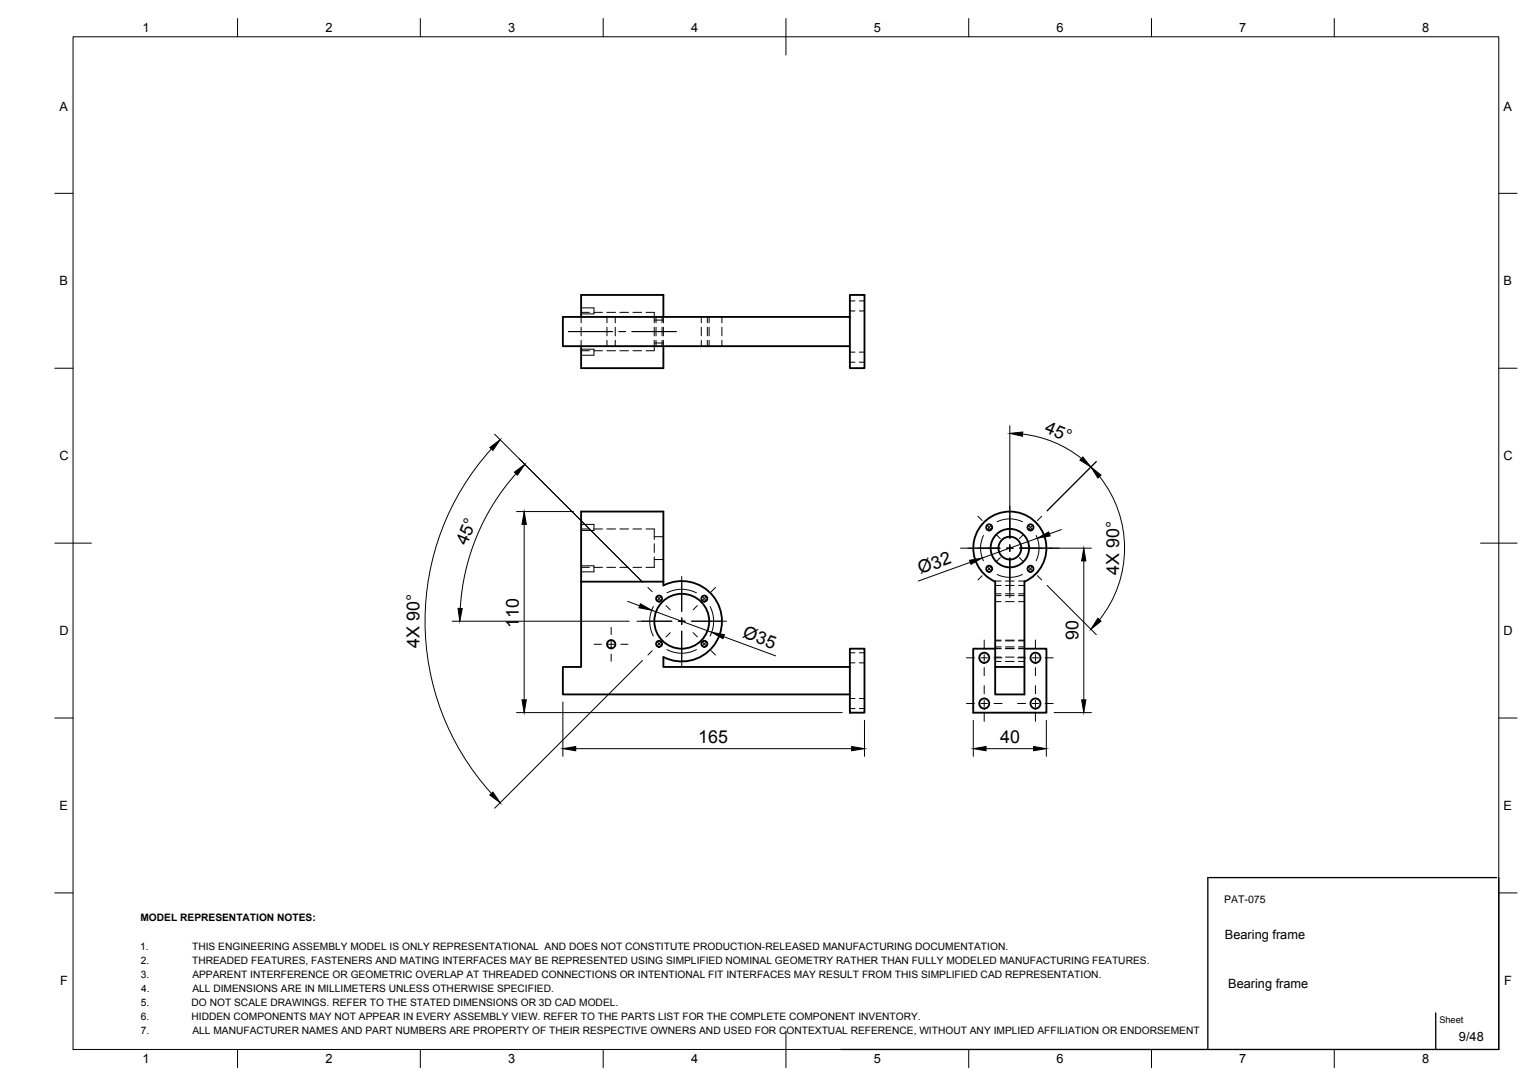
ISO-10303-21;
HEADER;
/* Generated by software containing ST-Developer
 * from STEP Tools, Inc. (www.steptools.com) 
 */

FILE_DESCRIPTION(
/* description */ ('Over-Centre Plunger Toggle Clamp on Slotted Fixture Frame'),
/* implementation_level */ '2;1');

FILE_NAME(
/* name */ 
'Bearing frame.step',
/* time_stamp */ '2026-10-28T03:23:24-07:00',
/* author */ (''),
/* organization */ (''),
/* preprocessor_version */ 'ST-DEVELOPER v20.2',
/* originating_system */ 'Autodesk Translation Framework v15.17.0.0',
/* authorisation */ '');

FILE_SCHEMA (('AUTOMOTIVE_DESIGN { 1 0 10303 214 3 1 1 }'));
ENDSEC;

DATA;
#10=MECHANICAL_DESIGN_GEOMETRIC_PRESENTATION_REPRESENTATION('',(#517),#15212);
#433=SHAPE_REPRESENTATION_RELATIONSHIP('SRR','None',#15407,#475);
#475=ADVANCED_BREP_SHAPE_REPRESENTATION('',(#568),#15169);
#517=STYLED_ITEM('',(#15719),#568);
#568=MANIFOLD_SOLID_BREP('Body1',#8249);
#643=FACE_BOUND('',#1664,.T.);
#644=FACE_BOUND('',#1669,.T.);
#645=FACE_BOUND('',#1670,.T.);
#646=FACE_BOUND('',#1671,.T.);
#647=FACE_BOUND('',#1672,.T.);
#648=FACE_BOUND('',#1673,.T.);
#649=FACE_BOUND('',#1674,.T.);
#650=FACE_BOUND('',#1676,.T.);
#651=FACE_BOUND('',#1677,.T.);
#652=FACE_BOUND('',#1678,.T.);
#653=FACE_BOUND('',#1679,.T.);
#654=FACE_BOUND('',#1680,.T.);
#655=FACE_BOUND('',#1682,.T.);
#656=FACE_BOUND('',#1683,.T.);
#657=FACE_BOUND('',#1684,.T.);
#658=FACE_BOUND('',#1685,.T.);
#659=FACE_BOUND('',#1686,.T.);
#660=FACE_BOUND('',#1694,.T.);
#661=FACE_BOUND('',#1695,.T.);
#662=FACE_BOUND('',#1696,.T.);
#663=FACE_BOUND('',#1697,.T.);
#664=FACE_BOUND('',#1698,.T.);
#665=FACE_BOUND('',#1699,.T.);
#666=FACE_BOUND('',#1702,.T.);
#667=FACE_BOUND('',#1707,.T.);
#668=FACE_BOUND('',#1708,.T.);
#669=FACE_BOUND('',#1709,.T.);
#670=FACE_BOUND('',#1710,.T.);
#807=PLANE('',#8848);
#808=PLANE('',#8852);
#809=PLANE('',#8856);
#810=PLANE('',#8860);
#811=PLANE('',#8888);
#812=PLANE('',#8898);
#813=PLANE('',#8900);
#814=PLANE('',#8901);
#815=PLANE('',#8902);
#816=PLANE('',#8903);
#817=PLANE('',#8904);
#818=PLANE('',#8905);
#819=PLANE('',#8906);
#820=PLANE('',#8909);
#821=PLANE('',#8910);
#822=PLANE('',#8911);
#823=PLANE('',#8912);
#824=PLANE('',#8913);
#825=PLANE('',#8914);
#826=PLANE('',#8915);
#1127=FACE_OUTER_BOUND('',#1645,.T.);
#1128=FACE_OUTER_BOUND('',#1646,.T.);
#1129=FACE_OUTER_BOUND('',#1647,.T.);
#1130=FACE_OUTER_BOUND('',#1648,.T.);
#1131=FACE_OUTER_BOUND('',#1649,.T.);
#1132=FACE_OUTER_BOUND('',#1650,.T.);
#1133=FACE_OUTER_BOUND('',#1651,.T.);
#1134=FACE_OUTER_BOUND('',#1652,.T.);
#1135=FACE_OUTER_BOUND('',#1653,.T.);
#1136=FACE_OUTER_BOUND('',#1654,.T.);
#1137=FACE_OUTER_BOUND('',#1655,.T.);
#1138=FACE_OUTER_BOUND('',#1656,.T.);
#1139=FACE_OUTER_BOUND('',#1657,.T.);
#1140=FACE_OUTER_BOUND('',#1658,.T.);
#1141=FACE_OUTER_BOUND('',#1659,.T.);
#1142=FACE_OUTER_BOUND('',#1660,.T.);
#1143=FACE_OUTER_BOUND('',#1661,.T.);
#1144=FACE_OUTER_BOUND('',#1662,.T.);
#1145=FACE_OUTER_BOUND('',#1663,.T.);
#1146=FACE_OUTER_BOUND('',#1665,.T.);
#1147=FACE_OUTER_BOUND('',#1666,.T.);
#1148=FACE_OUTER_BOUND('',#1667,.T.);
#1149=FACE_OUTER_BOUND('',#1668,.T.);
#1150=FACE_OUTER_BOUND('',#1675,.T.);
#1151=FACE_OUTER_BOUND('',#1681,.T.);
#1152=FACE_OUTER_BOUND('',#1687,.T.);
#1153=FACE_OUTER_BOUND('',#1688,.T.);
#1154=FACE_OUTER_BOUND('',#1689,.T.);
#1155=FACE_OUTER_BOUND('',#1690,.T.);
#1156=FACE_OUTER_BOUND('',#1691,.T.);
#1157=FACE_OUTER_BOUND('',#1692,.T.);
#1158=FACE_OUTER_BOUND('',#1693,.T.);
#1159=FACE_OUTER_BOUND('',#1700,.T.);
#1160=FACE_OUTER_BOUND('',#1701,.T.);
#1161=FACE_OUTER_BOUND('',#1703,.T.);
#1162=FACE_OUTER_BOUND('',#1704,.T.);
#1163=FACE_OUTER_BOUND('',#1705,.T.);
#1164=FACE_OUTER_BOUND('',#1706,.T.);
#1645=EDGE_LOOP('',(#5761,#5762,#5763,#5764));
#1646=EDGE_LOOP('',(#5765,#5766,#5767,#5768));
#1647=EDGE_LOOP('',(#5769));
#1648=EDGE_LOOP('',(#5770,#5771,#5772,#5773));
#1649=EDGE_LOOP('',(#5774));
#1650=EDGE_LOOP('',(#5775,#5776,#5777,#5778));
#1651=EDGE_LOOP('',(#5779));
#1652=EDGE_LOOP('',(#5780,#5781,#5782,#5783));
#1653=EDGE_LOOP('',(#5784));
#1654=EDGE_LOOP('',(#5785,#5786,#5787,#5788));
#1655=EDGE_LOOP('',(#5789,#5790,#5791,#5792));
#1656=EDGE_LOOP('',(#5793,#5794,#5795,#5796));
#1657=EDGE_LOOP('',(#5797,#5798,#5799,#5800));
#1658=EDGE_LOOP('',(#5801,#5802,#5803,#5804));
#1659=EDGE_LOOP('',(#5805,#5806,#5807,#5808));
#1660=EDGE_LOOP('',(#5809,#5810,#5811,#5812));
#1661=EDGE_LOOP('',(#5813,#5814,#5815,#5816));
#1662=EDGE_LOOP('',(#5817,#5818,#5819,#5820));
#1663=EDGE_LOOP('',(#5821));
#1664=EDGE_LOOP('',(#5822));
#1665=EDGE_LOOP('',(#5823,#5824,#5825,#5826));
#1666=EDGE_LOOP('',(#5827,#5828,#5829,#5830));
#1667=EDGE_LOOP('',(#5831,#5832,#5833,#5834));
#1668=EDGE_LOOP('',(#5835,#5836,#5837,#5838,#5839,#5840,#5841,#5842,#5843,
#5844));
#1669=EDGE_LOOP('',(#5845));
#1670=EDGE_LOOP('',(#5846));
#1671=EDGE_LOOP('',(#5847));
#1672=EDGE_LOOP('',(#5848));
#1673=EDGE_LOOP('',(#5849));
#1674=EDGE_LOOP('',(#5850));
#1675=EDGE_LOOP('',(#5851,#5852,#5853,#5854));
#1676=EDGE_LOOP('',(#5855));
#1677=EDGE_LOOP('',(#5856));
#1678=EDGE_LOOP('',(#5857));
#1679=EDGE_LOOP('',(#5858));
#1680=EDGE_LOOP('',(#5859));
#1681=EDGE_LOOP('',(#5860,#5861,#5862,#5863));
#1682=EDGE_LOOP('',(#5864,#5865,#5866,#5867));
#1683=EDGE_LOOP('',(#5868));
#1684=EDGE_LOOP('',(#5869));
#1685=EDGE_LOOP('',(#5870));
#1686=EDGE_LOOP('',(#5871));
#1687=EDGE_LOOP('',(#5872,#5873,#5874,#5875));
#1688=EDGE_LOOP('',(#5876,#5877,#5878,#5879));
#1689=EDGE_LOOP('',(#5880,#5881,#5882,#5883));
#1690=EDGE_LOOP('',(#5884,#5885,#5886,#5887));
#1691=EDGE_LOOP('',(#5888,#5889,#5890,#5891));
#1692=EDGE_LOOP('',(#5892,#5893,#5894,#5895));
#1693=EDGE_LOOP('',(#5896,#5897,#5898,#5899,#5900,#5901,#5902,#5903,#5904,
#5905));
#1694=EDGE_LOOP('',(#5906));
#1695=EDGE_LOOP('',(#5907));
#1696=EDGE_LOOP('',(#5908));
#1697=EDGE_LOOP('',(#5909));
#1698=EDGE_LOOP('',(#5910));
#1699=EDGE_LOOP('',(#5911));
#1700=EDGE_LOOP('',(#5912,#5913,#5914,#5915));
#1701=EDGE_LOOP('',(#5916,#5917,#5918,#5919));
#1702=EDGE_LOOP('',(#5920));
#1703=EDGE_LOOP('',(#5921,#5922,#5923,#5924));
#1704=EDGE_LOOP('',(#5925,#5926,#5927,#5928));
#1705=EDGE_LOOP('',(#5929,#5930,#5931,#5932));
#1706=EDGE_LOOP('',(#5933,#5934,#5935,#5936));
#1707=EDGE_LOOP('',(#5937));
#1708=EDGE_LOOP('',(#5938));
#1709=EDGE_LOOP('',(#5939));
#1710=EDGE_LOOP('',(#5940));
#2295=LINE('',#12577,#2925);
#2296=LINE('',#12583,#2926);
#2297=LINE('',#12590,#2927);
#2298=LINE('',#12597,#2928);
#2299=LINE('',#12604,#2929);
#2300=LINE('',#12611,#2930);
#2301=LINE('',#12617,#2931);
#2302=LINE('',#12623,#2932);
#2303=LINE('',#12629,#2933);
#2304=LINE('',#12635,#2934);
#2305=LINE('',#12641,#2935);
#2306=LINE('',#12647,#2936);
#2307=LINE('',#12653,#2937);
#2308=LINE('',#12659,#2938);
#2309=LINE('',#12667,#2939);
#2310=LINE('',#12672,#2940);
#2311=LINE('',#12677,#2941);
#2312=LINE('',#12681,#2942);
#2313=LINE('',#12685,#2943);
#2314=LINE('',#12687,#2944);
#2315=LINE('',#12689,#2945);
#2316=LINE('',#12691,#2946);
#2317=LINE('',#12693,#2947);
#2318=LINE('',#12695,#2948);
#2319=LINE('',#12697,#2949);
#2320=LINE('',#12700,#2950);
#2321=LINE('',#12703,#2951);
#2322=LINE('',#12704,#2952);
#2323=LINE('',#12708,#2953);
#2324=LINE('',#12710,#2954);
#2325=LINE('',#12712,#2955);
#2326=LINE('',#12713,#2956);
#2327=LINE('',#12716,#2957);
#2328=LINE('',#12717,#2958);
#2329=LINE('',#12718,#2959);
#2330=LINE('',#12722,#2960);
#2331=LINE('',#12723,#2961);
#2332=LINE('',#12724,#2962);
#2333=LINE('',#12727,#2963);
#2334=LINE('',#12728,#2964);
#2335=LINE('',#12731,#2965);
#2336=LINE('',#12732,#2966);
#2337=LINE('',#12734,#2967);
#2338=LINE('',#12737,#2968);
#2339=LINE('',#12738,#2969);
#2340=LINE('',#12741,#2970);
#2341=LINE('',#12743,#2971);
#2342=LINE('',#12746,#2972);
#2343=LINE('',#12747,#2973);
#2344=LINE('',#12749,#2974);
#2345=LINE('',#12751,#2975);
#2346=LINE('',#12752,#2976);
#2347=LINE('',#12756,#2977);
#2348=LINE('',#12758,#2978);
#2925=VECTOR('',#9980,0.225);
#2926=VECTOR('',#9987,0.165);
#2927=VECTOR('',#9996,0.165);
#2928=VECTOR('',#10005,0.165);
#2929=VECTOR('',#10014,0.165);
#2930=VECTOR('',#10023,0.165);
#2931=VECTOR('',#10030,0.165);
#2932=VECTOR('',#10037,0.165);
#2933=VECTOR('',#10044,0.165);
#2934=VECTOR('',#10051,0.275);
#2935=VECTOR('',#10058,0.275);
#2936=VECTOR('',#10065,0.275);
#2937=VECTOR('',#10072,0.275);
#2938=VECTOR('',#10079,1.05);
#2939=VECTOR('',#10090,0.625);
#2940=VECTOR('',#10095,1.5);
#2941=VECTOR('',#10100,1.);
#2942=VECTOR('',#10103,1.);
#2943=VECTOR('',#10108,1.);
#2944=VECTOR('',#10109,1.);
#2945=VECTOR('',#10110,1.);
#2946=VECTOR('',#10111,1.);
#2947=VECTOR('',#10112,1.);
#2948=VECTOR('',#10113,1.);
#2949=VECTOR('',#10114,1.);
#2950=VECTOR('',#10117,1.);
#2951=VECTOR('',#10120,1.);
#2952=VECTOR('',#10121,1.);
#2953=VECTOR('',#10124,1.);
#2954=VECTOR('',#10125,1.);
#2955=VECTOR('',#10126,1.);
#2956=VECTOR('',#10127,1.);
#2957=VECTOR('',#10128,1.);
#2958=VECTOR('',#10129,1.);
#2959=VECTOR('',#10130,1.);
#2960=VECTOR('',#10133,1.);
#2961=VECTOR('',#10134,1.);
#2962=VECTOR('',#10135,1.);
#2963=VECTOR('',#10138,1.);
#2964=VECTOR('',#10139,1.);
#2965=VECTOR('',#10142,1.);
#2966=VECTOR('',#10143,1.);
#2967=VECTOR('',#10146,1.);
#2968=VECTOR('',#10149,1.);
#2969=VECTOR('',#10150,1.);
#2970=VECTOR('',#10153,1.);
#2971=VECTOR('',#10154,1.);
#2972=VECTOR('',#10159,1.);
#2973=VECTOR('',#10160,1.);
#2974=VECTOR('',#10161,1.);
#2975=VECTOR('',#10162,1.);
#2976=VECTOR('',#10163,1.);
#2977=VECTOR('',#10170,1.);
#2978=VECTOR('',#10173,1.);
#3523=CIRCLE('',#8843,0.225);
#3524=CIRCLE('',#8844,0.225);
#3525=CIRCLE('',#8846,0.165);
#3526=CIRCLE('',#8847,0.165);
#3527=CIRCLE('',#8850,0.165);
#3528=CIRCLE('',#8851,0.165);
#3529=CIRCLE('',#8854,0.165);
#3530=CIRCLE('',#8855,0.165);
#3531=CIRCLE('',#8858,0.165);
#3532=CIRCLE('',#8859,0.165);
#3533=CIRCLE('',#8862,0.165);
#3534=CIRCLE('',#8863,0.165);
#3535=CIRCLE('',#8865,0.165);
#3536=CIRCLE('',#8866,0.165);
#3537=CIRCLE('',#8868,0.165);
#3538=CIRCLE('',#8869,0.165);
#3539=CIRCLE('',#8871,0.165);
#3540=CIRCLE('',#8872,0.165);
#3541=CIRCLE('',#8874,0.275);
#3542=CIRCLE('',#8875,0.275);
#3543=CIRCLE('',#8877,0.275);
#3544=CIRCLE('',#8878,0.275);
#3545=CIRCLE('',#8880,0.275);
#3546=CIRCLE('',#8881,0.275);
#3547=CIRCLE('',#8883,0.275);
#3548=CIRCLE('',#8884,0.275);
#3549=CIRCLE('',#8886,1.05);
#3550=CIRCLE('',#8887,1.05);
#3551=CIRCLE('',#8889,0.625);
#3552=CIRCLE('',#8891,0.625);
#3553=CIRCLE('',#8893,1.5);
#3554=CIRCLE('',#8894,1.5);
#3555=CIRCLE('',#8896,2.);
#3556=CIRCLE('',#8897,2.);
#3557=CIRCLE('',#8899,2.2);
#3558=CIRCLE('',#8908,2.2);
#3923=VERTEX_POINT('',#12574);
#3924=VERTEX_POINT('',#12576);
#3925=VERTEX_POINT('',#12580);
#3926=VERTEX_POINT('',#12582);
#3927=VERTEX_POINT('',#12587);
#3928=VERTEX_POINT('',#12589);
#3929=VERTEX_POINT('',#12594);
#3930=VERTEX_POINT('',#12596);
#3931=VERTEX_POINT('',#12601);
#3932=VERTEX_POINT('',#12603);
#3933=VERTEX_POINT('',#12608);
#3934=VERTEX_POINT('',#12610);
#3935=VERTEX_POINT('',#12614);
#3936=VERTEX_POINT('',#12616);
#3937=VERTEX_POINT('',#12620);
#3938=VERTEX_POINT('',#12622);
#3939=VERTEX_POINT('',#12626);
#3940=VERTEX_POINT('',#12628);
#3941=VERTEX_POINT('',#12632);
#3942=VERTEX_POINT('',#12634);
#3943=VERTEX_POINT('',#12638);
#3944=VERTEX_POINT('',#12640);
#3945=VERTEX_POINT('',#12644);
#3946=VERTEX_POINT('',#12646);
#3947=VERTEX_POINT('',#12650);
#3948=VERTEX_POINT('',#12652);
#3949=VERTEX_POINT('',#12656);
#3950=VERTEX_POINT('',#12658);
#3951=VERTEX_POINT('',#12662);
#3952=VERTEX_POINT('',#12665);
#3953=VERTEX_POINT('',#12669);
#3954=VERTEX_POINT('',#12671);
#3955=VERTEX_POINT('',#12675);
#3956=VERTEX_POINT('',#12676);
#3957=VERTEX_POINT('',#12678);
#3958=VERTEX_POINT('',#12680);
#3959=VERTEX_POINT('',#12684);
#3960=VERTEX_POINT('',#12686);
#3961=VERTEX_POINT('',#12688);
#3962=VERTEX_POINT('',#12690);
#3963=VERTEX_POINT('',#12692);
#3964=VERTEX_POINT('',#12694);
#3965=VERTEX_POINT('',#12696);
#3966=VERTEX_POINT('',#12698);
#3967=VERTEX_POINT('',#12702);
#3968=VERTEX_POINT('',#12706);
#3969=VERTEX_POINT('',#12707);
#3970=VERTEX_POINT('',#12709);
#3971=VERTEX_POINT('',#12711);
#3972=VERTEX_POINT('',#12714);
#3973=VERTEX_POINT('',#12715);
#3974=VERTEX_POINT('',#12720);
#3975=VERTEX_POINT('',#12721);
#3976=VERTEX_POINT('',#12726);
#3977=VERTEX_POINT('',#12730);
#3978=VERTEX_POINT('',#12736);
#3979=VERTEX_POINT('',#12740);
#3980=VERTEX_POINT('',#12742);
#3981=VERTEX_POINT('',#12748);
#3982=VERTEX_POINT('',#12750);
#4641=EDGE_CURVE('',#3923,#3923,#3523,.T.);
#4642=EDGE_CURVE('',#3923,#3924,#2295,.T.);
#4643=EDGE_CURVE('',#3924,#3924,#3524,.T.);
#4644=EDGE_CURVE('',#3925,#3925,#3525,.T.);
#4645=EDGE_CURVE('',#3925,#3926,#2296,.T.);
#4646=EDGE_CURVE('',#3926,#3926,#3526,.T.);
#4647=EDGE_CURVE('',#3927,#3927,#3527,.T.);
#4648=EDGE_CURVE('',#3927,#3928,#2297,.T.);
#4649=EDGE_CURVE('',#3928,#3928,#3528,.T.);
#4650=EDGE_CURVE('',#3929,#3929,#3529,.T.);
#4651=EDGE_CURVE('',#3929,#3930,#2298,.T.);
#4652=EDGE_CURVE('',#3930,#3930,#3530,.T.);
#4653=EDGE_CURVE('',#3931,#3931,#3531,.T.);
#4654=EDGE_CURVE('',#3931,#3932,#2299,.T.);
#4655=EDGE_CURVE('',#3932,#3932,#3532,.T.);
#4656=EDGE_CURVE('',#3933,#3933,#3533,.T.);
#4657=EDGE_CURVE('',#3933,#3934,#2300,.T.);
#4658=EDGE_CURVE('',#3934,#3934,#3534,.T.);
#4659=EDGE_CURVE('',#3935,#3935,#3535,.T.);
#4660=EDGE_CURVE('',#3935,#3936,#2301,.T.);
#4661=EDGE_CURVE('',#3936,#3936,#3536,.T.);
#4662=EDGE_CURVE('',#3937,#3937,#3537,.T.);
#4663=EDGE_CURVE('',#3937,#3938,#2302,.T.);
#4664=EDGE_CURVE('',#3938,#3938,#3538,.T.);
#4665=EDGE_CURVE('',#3939,#3939,#3539,.T.);
#4666=EDGE_CURVE('',#3939,#3940,#2303,.T.);
#4667=EDGE_CURVE('',#3940,#3940,#3540,.T.);
#4668=EDGE_CURVE('',#3941,#3941,#3541,.T.);
#4669=EDGE_CURVE('',#3941,#3942,#2304,.T.);
#4670=EDGE_CURVE('',#3942,#3942,#3542,.T.);
#4671=EDGE_CURVE('',#3943,#3943,#3543,.T.);
#4672=EDGE_CURVE('',#3943,#3944,#2305,.T.);
#4673=EDGE_CURVE('',#3944,#3944,#3544,.T.);
#4674=EDGE_CURVE('',#3945,#3945,#3545,.T.);
#4675=EDGE_CURVE('',#3945,#3946,#2306,.T.);
#4676=EDGE_CURVE('',#3946,#3946,#3546,.T.);
#4677=EDGE_CURVE('',#3947,#3947,#3547,.T.);
#4678=EDGE_CURVE('',#3947,#3948,#2307,.T.);
#4679=EDGE_CURVE('',#3948,#3948,#3548,.T.);
#4680=EDGE_CURVE('',#3949,#3949,#3549,.T.);
#4681=EDGE_CURVE('',#3949,#3950,#2308,.T.);
#4682=EDGE_CURVE('',#3950,#3950,#3550,.T.);
#4683=EDGE_CURVE('',#3951,#3951,#3551,.T.);
#4684=EDGE_CURVE('',#3952,#3952,#3552,.T.);
#4685=EDGE_CURVE('',#3952,#3951,#2309,.T.);
#4686=EDGE_CURVE('',#3953,#3953,#3553,.T.);
#4687=EDGE_CURVE('',#3953,#3954,#2310,.T.);
#4688=EDGE_CURVE('',#3954,#3954,#3554,.T.);
#4689=EDGE_CURVE('',#3955,#3956,#2311,.T.);
#4690=EDGE_CURVE('',#3955,#3957,#3555,.T.);
#4691=EDGE_CURVE('',#3958,#3957,#2312,.T.);
#4692=EDGE_CURVE('',#3956,#3958,#3556,.T.);
#4693=EDGE_CURVE('',#3956,#3959,#2313,.T.);
#4694=EDGE_CURVE('',#3959,#3960,#2314,.T.);
#4695=EDGE_CURVE('',#3961,#3960,#2315,.T.);
#4696=EDGE_CURVE('',#3962,#3961,#2316,.T.);
#4697=EDGE_CURVE('',#3962,#3963,#2317,.T.);
#4698=EDGE_CURVE('',#3963,#3964,#2318,.T.);
#4699=EDGE_CURVE('',#3964,#3965,#2319,.T.);
#4700=EDGE_CURVE('',#3966,#3965,#3557,.T.);
#4701=EDGE_CURVE('',#3966,#3955,#2320,.T.);
#4702=EDGE_CURVE('',#3967,#3958,#2321,.T.);
#4703=EDGE_CURVE('',#3959,#3967,#2322,.T.);
#4704=EDGE_CURVE('',#3968,#3969,#2323,.T.);
#4705=EDGE_CURVE('',#3969,#3970,#2324,.T.);
#4706=EDGE_CURVE('',#3970,#3971,#2325,.T.);
#4707=EDGE_CURVE('',#3971,#3968,#2326,.T.);
#4708=EDGE_CURVE('',#3972,#3973,#2327,.T.);
#4709=EDGE_CURVE('',#3963,#3972,#2328,.T.);
#4710=EDGE_CURVE('',#3973,#3962,#2329,.T.);
#4711=EDGE_CURVE('',#3974,#3975,#2330,.T.);
#4712=EDGE_CURVE('',#3975,#3968,#2331,.T.);
#4713=EDGE_CURVE('',#3974,#3971,#2332,.T.);
#4714=EDGE_CURVE('',#3976,#3974,#2333,.T.);
#4715=EDGE_CURVE('',#3976,#3970,#2334,.T.);
#4716=EDGE_CURVE('',#3977,#3976,#2335,.T.);
#4717=EDGE_CURVE('',#3977,#3969,#2336,.T.);
#4718=EDGE_CURVE('',#3975,#3977,#2337,.T.);
#4719=EDGE_CURVE('',#3972,#3978,#2338,.T.);
#4720=EDGE_CURVE('',#3978,#3964,#2339,.T.);
#4721=EDGE_CURVE('',#3966,#3979,#2340,.T.);
#4722=EDGE_CURVE('',#3980,#3965,#2341,.T.);
#4723=EDGE_CURVE('',#3979,#3980,#3558,.T.);
#4724=EDGE_CURVE('',#3957,#3979,#2342,.T.);
#4725=EDGE_CURVE('',#3980,#3978,#2343,.T.);
#4726=EDGE_CURVE('',#3973,#3981,#2344,.T.);
#4727=EDGE_CURVE('',#3982,#3981,#2345,.T.);
#4728=EDGE_CURVE('',#3967,#3982,#2346,.T.);
#4729=EDGE_CURVE('',#3960,#3982,#2347,.T.);
#4730=EDGE_CURVE('',#3981,#3961,#2348,.T.);
#5761=ORIENTED_EDGE('',*,*,#4641,.F.);
#5762=ORIENTED_EDGE('',*,*,#4642,.T.);
#5763=ORIENTED_EDGE('',*,*,#4643,.F.);
#5764=ORIENTED_EDGE('',*,*,#4642,.F.);
#5765=ORIENTED_EDGE('',*,*,#4644,.F.);
#5766=ORIENTED_EDGE('',*,*,#4645,.T.);
#5767=ORIENTED_EDGE('',*,*,#4646,.F.);
#5768=ORIENTED_EDGE('',*,*,#4645,.F.);
#5769=ORIENTED_EDGE('',*,*,#4644,.T.);
#5770=ORIENTED_EDGE('',*,*,#4647,.F.);
#5771=ORIENTED_EDGE('',*,*,#4648,.T.);
#5772=ORIENTED_EDGE('',*,*,#4649,.F.);
#5773=ORIENTED_EDGE('',*,*,#4648,.F.);
#5774=ORIENTED_EDGE('',*,*,#4647,.T.);
#5775=ORIENTED_EDGE('',*,*,#4650,.F.);
#5776=ORIENTED_EDGE('',*,*,#4651,.T.);
#5777=ORIENTED_EDGE('',*,*,#4652,.F.);
#5778=ORIENTED_EDGE('',*,*,#4651,.F.);
#5779=ORIENTED_EDGE('',*,*,#4650,.T.);
#5780=ORIENTED_EDGE('',*,*,#4653,.F.);
#5781=ORIENTED_EDGE('',*,*,#4654,.T.);
#5782=ORIENTED_EDGE('',*,*,#4655,.F.);
#5783=ORIENTED_EDGE('',*,*,#4654,.F.);
#5784=ORIENTED_EDGE('',*,*,#4653,.T.);
#5785=ORIENTED_EDGE('',*,*,#4656,.F.);
#5786=ORIENTED_EDGE('',*,*,#4657,.T.);
#5787=ORIENTED_EDGE('',*,*,#4658,.F.);
#5788=ORIENTED_EDGE('',*,*,#4657,.F.);
#5789=ORIENTED_EDGE('',*,*,#4659,.F.);
#5790=ORIENTED_EDGE('',*,*,#4660,.T.);
#5791=ORIENTED_EDGE('',*,*,#4661,.F.);
#5792=ORIENTED_EDGE('',*,*,#4660,.F.);
#5793=ORIENTED_EDGE('',*,*,#4662,.F.);
#5794=ORIENTED_EDGE('',*,*,#4663,.T.);
#5795=ORIENTED_EDGE('',*,*,#4664,.F.);
#5796=ORIENTED_EDGE('',*,*,#4663,.F.);
#5797=ORIENTED_EDGE('',*,*,#4665,.F.);
#5798=ORIENTED_EDGE('',*,*,#4666,.T.);
#5799=ORIENTED_EDGE('',*,*,#4667,.F.);
#5800=ORIENTED_EDGE('',*,*,#4666,.F.);
#5801=ORIENTED_EDGE('',*,*,#4668,.F.);
#5802=ORIENTED_EDGE('',*,*,#4669,.T.);
#5803=ORIENTED_EDGE('',*,*,#4670,.F.);
#5804=ORIENTED_EDGE('',*,*,#4669,.F.);
#5805=ORIENTED_EDGE('',*,*,#4671,.F.);
#5806=ORIENTED_EDGE('',*,*,#4672,.T.);
#5807=ORIENTED_EDGE('',*,*,#4673,.F.);
#5808=ORIENTED_EDGE('',*,*,#4672,.F.);
#5809=ORIENTED_EDGE('',*,*,#4674,.F.);
#5810=ORIENTED_EDGE('',*,*,#4675,.T.);
#5811=ORIENTED_EDGE('',*,*,#4676,.F.);
#5812=ORIENTED_EDGE('',*,*,#4675,.F.);
#5813=ORIENTED_EDGE('',*,*,#4677,.F.);
#5814=ORIENTED_EDGE('',*,*,#4678,.T.);
#5815=ORIENTED_EDGE('',*,*,#4679,.F.);
#5816=ORIENTED_EDGE('',*,*,#4678,.F.);
#5817=ORIENTED_EDGE('',*,*,#4680,.F.);
#5818=ORIENTED_EDGE('',*,*,#4681,.T.);
#5819=ORIENTED_EDGE('',*,*,#4682,.F.);
#5820=ORIENTED_EDGE('',*,*,#4681,.F.);
#5821=ORIENTED_EDGE('',*,*,#4680,.T.);
#5822=ORIENTED_EDGE('',*,*,#4683,.F.);
#5823=ORIENTED_EDGE('',*,*,#4684,.F.);
#5824=ORIENTED_EDGE('',*,*,#4685,.T.);
#5825=ORIENTED_EDGE('',*,*,#4683,.T.);
#5826=ORIENTED_EDGE('',*,*,#4685,.F.);
#5827=ORIENTED_EDGE('',*,*,#4686,.F.);
#5828=ORIENTED_EDGE('',*,*,#4687,.T.);
#5829=ORIENTED_EDGE('',*,*,#4688,.F.);
#5830=ORIENTED_EDGE('',*,*,#4687,.F.);
#5831=ORIENTED_EDGE('',*,*,#4689,.F.);
#5832=ORIENTED_EDGE('',*,*,#4690,.T.);
#5833=ORIENTED_EDGE('',*,*,#4691,.F.);
#5834=ORIENTED_EDGE('',*,*,#4692,.F.);
#5835=ORIENTED_EDGE('',*,*,#4689,.T.);
#5836=ORIENTED_EDGE('',*,*,#4693,.T.);
#5837=ORIENTED_EDGE('',*,*,#4694,.T.);
#5838=ORIENTED_EDGE('',*,*,#4695,.F.);
#5839=ORIENTED_EDGE('',*,*,#4696,.F.);
#5840=ORIENTED_EDGE('',*,*,#4697,.T.);
#5841=ORIENTED_EDGE('',*,*,#4698,.T.);
#5842=ORIENTED_EDGE('',*,*,#4699,.T.);
#5843=ORIENTED_EDGE('',*,*,#4700,.F.);
#5844=ORIENTED_EDGE('',*,*,#4701,.T.);
#5845=ORIENTED_EDGE('',*,*,#4641,.T.);
#5846=ORIENTED_EDGE('',*,*,#4686,.T.);
#5847=ORIENTED_EDGE('',*,*,#4665,.T.);
#5848=ORIENTED_EDGE('',*,*,#4662,.T.);
#5849=ORIENTED_EDGE('',*,*,#4659,.T.);
#5850=ORIENTED_EDGE('',*,*,#4656,.T.);
#5851=ORIENTED_EDGE('',*,*,#4692,.T.);
#5852=ORIENTED_EDGE('',*,*,#4702,.F.);
#5853=ORIENTED_EDGE('',*,*,#4703,.F.);
#5854=ORIENTED_EDGE('',*,*,#4693,.F.);
#5855=ORIENTED_EDGE('',*,*,#4682,.T.);
#5856=ORIENTED_EDGE('',*,*,#4655,.T.);
#5857=ORIENTED_EDGE('',*,*,#4652,.T.);
#5858=ORIENTED_EDGE('',*,*,#4649,.T.);
#5859=ORIENTED_EDGE('',*,*,#4646,.T.);
#5860=ORIENTED_EDGE('',*,*,#4704,.T.);
#5861=ORIENTED_EDGE('',*,*,#4705,.T.);
#5862=ORIENTED_EDGE('',*,*,#4706,.T.);
#5863=ORIENTED_EDGE('',*,*,#4707,.T.);
#5864=ORIENTED_EDGE('',*,*,#4708,.F.);
#5865=ORIENTED_EDGE('',*,*,#4709,.F.);
#5866=ORIENTED_EDGE('',*,*,#4697,.F.);
#5867=ORIENTED_EDGE('',*,*,#4710,.F.);
#5868=ORIENTED_EDGE('',*,*,#4679,.T.);
#5869=ORIENTED_EDGE('',*,*,#4676,.T.);
#5870=ORIENTED_EDGE('',*,*,#4673,.T.);
#5871=ORIENTED_EDGE('',*,*,#4670,.T.);
#5872=ORIENTED_EDGE('',*,*,#4711,.T.);
#5873=ORIENTED_EDGE('',*,*,#4712,.T.);
#5874=ORIENTED_EDGE('',*,*,#4707,.F.);
#5875=ORIENTED_EDGE('',*,*,#4713,.F.);
#5876=ORIENTED_EDGE('',*,*,#4714,.T.);
#5877=ORIENTED_EDGE('',*,*,#4713,.T.);
#5878=ORIENTED_EDGE('',*,*,#4706,.F.);
#5879=ORIENTED_EDGE('',*,*,#4715,.F.);
#5880=ORIENTED_EDGE('',*,*,#4716,.T.);
#5881=ORIENTED_EDGE('',*,*,#4715,.T.);
#5882=ORIENTED_EDGE('',*,*,#4705,.F.);
#5883=ORIENTED_EDGE('',*,*,#4717,.F.);
#5884=ORIENTED_EDGE('',*,*,#4718,.T.);
#5885=ORIENTED_EDGE('',*,*,#4717,.T.);
#5886=ORIENTED_EDGE('',*,*,#4704,.F.);
#5887=ORIENTED_EDGE('',*,*,#4712,.F.);
#5888=ORIENTED_EDGE('',*,*,#4709,.T.);
#5889=ORIENTED_EDGE('',*,*,#4719,.T.);
#5890=ORIENTED_EDGE('',*,*,#4720,.T.);
#5891=ORIENTED_EDGE('',*,*,#4698,.F.);
#5892=ORIENTED_EDGE('',*,*,#4721,.F.);
#5893=ORIENTED_EDGE('',*,*,#4700,.T.);
#5894=ORIENTED_EDGE('',*,*,#4722,.F.);
#5895=ORIENTED_EDGE('',*,*,#4723,.F.);
#5896=ORIENTED_EDGE('',*,*,#4691,.T.);
#5897=ORIENTED_EDGE('',*,*,#4724,.T.);
#5898=ORIENTED_EDGE('',*,*,#4723,.T.);
#5899=ORIENTED_EDGE('',*,*,#4725,.T.);
#5900=ORIENTED_EDGE('',*,*,#4719,.F.);
#5901=ORIENTED_EDGE('',*,*,#4708,.T.);
#5902=ORIENTED_EDGE('',*,*,#4726,.T.);
#5903=ORIENTED_EDGE('',*,*,#4727,.F.);
#5904=ORIENTED_EDGE('',*,*,#4728,.F.);
#5905=ORIENTED_EDGE('',*,*,#4702,.T.);
#5906=ORIENTED_EDGE('',*,*,#4643,.T.);
#5907=ORIENTED_EDGE('',*,*,#4688,.T.);
#5908=ORIENTED_EDGE('',*,*,#4667,.T.);
#5909=ORIENTED_EDGE('',*,*,#4664,.T.);
#5910=ORIENTED_EDGE('',*,*,#4661,.T.);
#5911=ORIENTED_EDGE('',*,*,#4658,.T.);
#5912=ORIENTED_EDGE('',*,*,#4722,.T.);
#5913=ORIENTED_EDGE('',*,*,#4699,.F.);
#5914=ORIENTED_EDGE('',*,*,#4720,.F.);
#5915=ORIENTED_EDGE('',*,*,#4725,.F.);
#5916=ORIENTED_EDGE('',*,*,#4701,.F.);
#5917=ORIENTED_EDGE('',*,*,#4721,.T.);
#5918=ORIENTED_EDGE('',*,*,#4724,.F.);
#5919=ORIENTED_EDGE('',*,*,#4690,.F.);
#5920=ORIENTED_EDGE('',*,*,#4684,.T.);
#5921=ORIENTED_EDGE('',*,*,#4703,.T.);
#5922=ORIENTED_EDGE('',*,*,#4728,.T.);
#5923=ORIENTED_EDGE('',*,*,#4729,.F.);
#5924=ORIENTED_EDGE('',*,*,#4694,.F.);
#5925=ORIENTED_EDGE('',*,*,#4710,.T.);
#5926=ORIENTED_EDGE('',*,*,#4696,.T.);
#5927=ORIENTED_EDGE('',*,*,#4730,.F.);
#5928=ORIENTED_EDGE('',*,*,#4726,.F.);
#5929=ORIENTED_EDGE('',*,*,#4730,.T.);
#5930=ORIENTED_EDGE('',*,*,#4695,.T.);
#5931=ORIENTED_EDGE('',*,*,#4729,.T.);
#5932=ORIENTED_EDGE('',*,*,#4727,.T.);
#5933=ORIENTED_EDGE('',*,*,#4718,.F.);
#5934=ORIENTED_EDGE('',*,*,#4711,.F.);
#5935=ORIENTED_EDGE('',*,*,#4714,.F.);
#5936=ORIENTED_EDGE('',*,*,#4716,.F.);
#5937=ORIENTED_EDGE('',*,*,#4668,.T.);
#5938=ORIENTED_EDGE('',*,*,#4671,.T.);
#5939=ORIENTED_EDGE('',*,*,#4674,.T.);
#5940=ORIENTED_EDGE('',*,*,#4677,.T.);
#7633=CYLINDRICAL_SURFACE('',#8842,0.225);
#7634=CYLINDRICAL_SURFACE('',#8845,0.165);
#7635=CYLINDRICAL_SURFACE('',#8849,0.165);
#7636=CYLINDRICAL_SURFACE('',#8853,0.165);
#7637=CYLINDRICAL_SURFACE('',#8857,0.165);
#7638=CYLINDRICAL_SURFACE('',#8861,0.165);
#7639=CYLINDRICAL_SURFACE('',#8864,0.165);
#7640=CYLINDRICAL_SURFACE('',#8867,0.165);
#7641=CYLINDRICAL_SURFACE('',#8870,0.165);
#7642=CYLINDRICAL_SURFACE('',#8873,0.275);
#7643=CYLINDRICAL_SURFACE('',#8876,0.275);
#7644=CYLINDRICAL_SURFACE('',#8879,0.275);
#7645=CYLINDRICAL_SURFACE('',#8882,0.275);
#7646=CYLINDRICAL_SURFACE('',#8885,1.05);
#7647=CYLINDRICAL_SURFACE('',#8890,0.625);
#7648=CYLINDRICAL_SURFACE('',#8892,1.5);
#7649=CYLINDRICAL_SURFACE('',#8895,2.);
#7650=CYLINDRICAL_SURFACE('',#8907,2.2);
#7799=ADVANCED_FACE('',(#1127),#7633,.F.);
#7800=ADVANCED_FACE('',(#1128),#7634,.F.);
#7801=ADVANCED_FACE('',(#1129),#807,.T.);
#7802=ADVANCED_FACE('',(#1130),#7635,.F.);
#7803=ADVANCED_FACE('',(#1131),#808,.T.);
#7804=ADVANCED_FACE('',(#1132),#7636,.F.);
#7805=ADVANCED_FACE('',(#1133),#809,.T.);
#7806=ADVANCED_FACE('',(#1134),#7637,.F.);
#7807=ADVANCED_FACE('',(#1135),#810,.T.);
#7808=ADVANCED_FACE('',(#1136),#7638,.F.);
#7809=ADVANCED_FACE('',(#1137),#7639,.F.);
#7810=ADVANCED_FACE('',(#1138),#7640,.F.);
#7811=ADVANCED_FACE('',(#1139),#7641,.F.);
#7812=ADVANCED_FACE('',(#1140),#7642,.F.);
#7813=ADVANCED_FACE('',(#1141),#7643,.F.);
#7814=ADVANCED_FACE('',(#1142),#7644,.F.);
#7815=ADVANCED_FACE('',(#1143),#7645,.F.);
#7816=ADVANCED_FACE('',(#1144),#7646,.F.);
#7817=ADVANCED_FACE('',(#1145,#643),#811,.T.);
#7818=ADVANCED_FACE('',(#1146),#7647,.F.);
#7819=ADVANCED_FACE('',(#1147),#7648,.F.);
#7820=ADVANCED_FACE('',(#1148),#7649,.T.);
#7821=ADVANCED_FACE('',(#1149,#644,#645,#646,#647,#648,#649),#812,.T.);
#7822=ADVANCED_FACE('',(#1150,#650,#651,#652,#653,#654),#813,.T.);
#7823=ADVANCED_FACE('',(#1151,#655,#656,#657,#658,#659),#814,.T.);
#7824=ADVANCED_FACE('',(#1152),#815,.T.);
#7825=ADVANCED_FACE('',(#1153),#816,.T.);
#7826=ADVANCED_FACE('',(#1154),#817,.T.);
#7827=ADVANCED_FACE('',(#1155),#818,.T.);
#7828=ADVANCED_FACE('',(#1156),#819,.T.);
#7829=ADVANCED_FACE('',(#1157),#7650,.T.);
#7830=ADVANCED_FACE('',(#1158,#660,#661,#662,#663,#664,#665),#820,.T.);
#7831=ADVANCED_FACE('',(#1159),#821,.T.);
#7832=ADVANCED_FACE('',(#1160,#666),#822,.T.);
#7833=ADVANCED_FACE('',(#1161),#823,.T.);
#7834=ADVANCED_FACE('',(#1162),#824,.T.);
#7835=ADVANCED_FACE('',(#1163),#825,.T.);
#7836=ADVANCED_FACE('',(#1164,#667,#668,#669,#670),#826,.F.);
#8249=CLOSED_SHELL('',(#7799,#7800,#7801,#7802,#7803,#7804,#7805,#7806,
#7807,#7808,#7809,#7810,#7811,#7812,#7813,#7814,#7815,#7816,#7817,#7818,
#7819,#7820,#7821,#7822,#7823,#7824,#7825,#7826,#7827,#7828,#7829,#7830,
#7831,#7832,#7833,#7834,#7835,#7836));
#8841=AXIS2_PLACEMENT_3D('',#12572,#9974,#9975);
#8842=AXIS2_PLACEMENT_3D('',#12573,#9976,#9977);
#8843=AXIS2_PLACEMENT_3D('',#12575,#9978,#9979);
#8844=AXIS2_PLACEMENT_3D('',#12578,#9981,#9982);
#8845=AXIS2_PLACEMENT_3D('',#12579,#9983,#9984);
#8846=AXIS2_PLACEMENT_3D('',#12581,#9985,#9986);
#8847=AXIS2_PLACEMENT_3D('',#12584,#9988,#9989);
#8848=AXIS2_PLACEMENT_3D('',#12585,#9990,#9991);
#8849=AXIS2_PLACEMENT_3D('',#12586,#9992,#9993);
#8850=AXIS2_PLACEMENT_3D('',#12588,#9994,#9995);
#8851=AXIS2_PLACEMENT_3D('',#12591,#9997,#9998);
#8852=AXIS2_PLACEMENT_3D('',#12592,#9999,#10000);
#8853=AXIS2_PLACEMENT_3D('',#12593,#10001,#10002);
#8854=AXIS2_PLACEMENT_3D('',#12595,#10003,#10004);
#8855=AXIS2_PLACEMENT_3D('',#12598,#10006,#10007);
#8856=AXIS2_PLACEMENT_3D('',#12599,#10008,#10009);
#8857=AXIS2_PLACEMENT_3D('',#12600,#10010,#10011);
#8858=AXIS2_PLACEMENT_3D('',#12602,#10012,#10013);
#8859=AXIS2_PLACEMENT_3D('',#12605,#10015,#10016);
#8860=AXIS2_PLACEMENT_3D('',#12606,#10017,#10018);
#8861=AXIS2_PLACEMENT_3D('',#12607,#10019,#10020);
#8862=AXIS2_PLACEMENT_3D('',#12609,#10021,#10022);
#8863=AXIS2_PLACEMENT_3D('',#12612,#10024,#10025);
#8864=AXIS2_PLACEMENT_3D('',#12613,#10026,#10027);
#8865=AXIS2_PLACEMENT_3D('',#12615,#10028,#10029);
#8866=AXIS2_PLACEMENT_3D('',#12618,#10031,#10032);
#8867=AXIS2_PLACEMENT_3D('',#12619,#10033,#10034);
#8868=AXIS2_PLACEMENT_3D('',#12621,#10035,#10036);
#8869=AXIS2_PLACEMENT_3D('',#12624,#10038,#10039);
#8870=AXIS2_PLACEMENT_3D('',#12625,#10040,#10041);
#8871=AXIS2_PLACEMENT_3D('',#12627,#10042,#10043);
#8872=AXIS2_PLACEMENT_3D('',#12630,#10045,#10046);
#8873=AXIS2_PLACEMENT_3D('',#12631,#10047,#10048);
#8874=AXIS2_PLACEMENT_3D('',#12633,#10049,#10050);
#8875=AXIS2_PLACEMENT_3D('',#12636,#10052,#10053);
#8876=AXIS2_PLACEMENT_3D('',#12637,#10054,#10055);
#8877=AXIS2_PLACEMENT_3D('',#12639,#10056,#10057);
#8878=AXIS2_PLACEMENT_3D('',#12642,#10059,#10060);
#8879=AXIS2_PLACEMENT_3D('',#12643,#10061,#10062);
#8880=AXIS2_PLACEMENT_3D('',#12645,#10063,#10064);
#8881=AXIS2_PLACEMENT_3D('',#12648,#10066,#10067);
#8882=AXIS2_PLACEMENT_3D('',#12649,#10068,#10069);
#8883=AXIS2_PLACEMENT_3D('',#12651,#10070,#10071);
#8884=AXIS2_PLACEMENT_3D('',#12654,#10073,#10074);
#8885=AXIS2_PLACEMENT_3D('',#12655,#10075,#10076);
#8886=AXIS2_PLACEMENT_3D('',#12657,#10077,#10078);
#8887=AXIS2_PLACEMENT_3D('',#12660,#10080,#10081);
#8888=AXIS2_PLACEMENT_3D('',#12661,#10082,#10083);
#8889=AXIS2_PLACEMENT_3D('',#12663,#10084,#10085);
#8890=AXIS2_PLACEMENT_3D('',#12664,#10086,#10087);
#8891=AXIS2_PLACEMENT_3D('',#12666,#10088,#10089);
#8892=AXIS2_PLACEMENT_3D('',#12668,#10091,#10092);
#8893=AXIS2_PLACEMENT_3D('',#12670,#10093,#10094);
#8894=AXIS2_PLACEMENT_3D('',#12673,#10096,#10097);
#8895=AXIS2_PLACEMENT_3D('',#12674,#10098,#10099);
#8896=AXIS2_PLACEMENT_3D('',#12679,#10101,#10102);
#8897=AXIS2_PLACEMENT_3D('',#12682,#10104,#10105);
#8898=AXIS2_PLACEMENT_3D('',#12683,#10106,#10107);
#8899=AXIS2_PLACEMENT_3D('',#12699,#10115,#10116);
#8900=AXIS2_PLACEMENT_3D('',#12701,#10118,#10119);
#8901=AXIS2_PLACEMENT_3D('',#12705,#10122,#10123);
#8902=AXIS2_PLACEMENT_3D('',#12719,#10131,#10132);
#8903=AXIS2_PLACEMENT_3D('',#12725,#10136,#10137);
#8904=AXIS2_PLACEMENT_3D('',#12729,#10140,#10141);
#8905=AXIS2_PLACEMENT_3D('',#12733,#10144,#10145);
#8906=AXIS2_PLACEMENT_3D('',#12735,#10147,#10148);
#8907=AXIS2_PLACEMENT_3D('',#12739,#10151,#10152);
#8908=AXIS2_PLACEMENT_3D('',#12744,#10155,#10156);
#8909=AXIS2_PLACEMENT_3D('',#12745,#10157,#10158);
#8910=AXIS2_PLACEMENT_3D('',#12753,#10164,#10165);
#8911=AXIS2_PLACEMENT_3D('',#12754,#10166,#10167);
#8912=AXIS2_PLACEMENT_3D('',#12755,#10168,#10169);
#8913=AXIS2_PLACEMENT_3D('',#12757,#10171,#10172);
#8914=AXIS2_PLACEMENT_3D('',#12759,#10174,#10175);
#8915=AXIS2_PLACEMENT_3D('',#12760,#10176,#10177);
#9974=DIRECTION('axis',(0.,0.,1.));
#9975=DIRECTION('refdir',(1.,0.,0.));
#9976=DIRECTION('center_axis',(0.,1.,0.));
#9977=DIRECTION('ref_axis',(1.,0.,0.));
#9978=DIRECTION('center_axis',(0.,1.,0.));
#9979=DIRECTION('ref_axis',(1.,0.,0.));
#9980=DIRECTION('',(0.,1.,0.));
#9981=DIRECTION('center_axis',(0.,-1.,0.));
#9982=DIRECTION('ref_axis',(1.,0.,0.));
#9983=DIRECTION('center_axis',(0.,0.,1.));
#9984=DIRECTION('ref_axis',(1.,0.,0.));
#9985=DIRECTION('center_axis',(0.,0.,1.));
#9986=DIRECTION('ref_axis',(1.,0.,0.));
#9987=DIRECTION('',(0.,0.,1.));
#9988=DIRECTION('center_axis',(0.,0.,-1.));
#9989=DIRECTION('ref_axis',(1.,0.,0.));
#9990=DIRECTION('center_axis',(0.,0.,1.));
#9991=DIRECTION('ref_axis',(1.,0.,0.));
#9992=DIRECTION('center_axis',(0.,0.,1.));
#9993=DIRECTION('ref_axis',(1.,0.,0.));
#9994=DIRECTION('center_axis',(0.,0.,1.));
#9995=DIRECTION('ref_axis',(1.,0.,0.));
#9996=DIRECTION('',(0.,0.,1.));
#9997=DIRECTION('center_axis',(0.,0.,-1.));
#9998=DIRECTION('ref_axis',(1.,0.,0.));
#9999=DIRECTION('center_axis',(0.,0.,1.));
#10000=DIRECTION('ref_axis',(1.,0.,0.));
#10001=DIRECTION('center_axis',(0.,0.,1.));
#10002=DIRECTION('ref_axis',(1.,0.,0.));
#10003=DIRECTION('center_axis',(0.,0.,1.));
#10004=DIRECTION('ref_axis',(1.,0.,0.));
#10005=DIRECTION('',(0.,0.,1.));
#10006=DIRECTION('center_axis',(0.,0.,-1.));
#10007=DIRECTION('ref_axis',(1.,0.,0.));
#10008=DIRECTION('center_axis',(0.,0.,1.));
#10009=DIRECTION('ref_axis',(1.,0.,0.));
#10010=DIRECTION('center_axis',(0.,0.,1.));
#10011=DIRECTION('ref_axis',(1.,0.,0.));
#10012=DIRECTION('center_axis',(0.,0.,1.));
#10013=DIRECTION('ref_axis',(1.,0.,0.));
#10014=DIRECTION('',(0.,0.,1.));
#10015=DIRECTION('center_axis',(0.,0.,-1.));
#10016=DIRECTION('ref_axis',(1.,0.,0.));
#10017=DIRECTION('center_axis',(0.,0.,1.));
#10018=DIRECTION('ref_axis',(1.,0.,0.));
#10019=DIRECTION('center_axis',(0.,1.,0.));
#10020=DIRECTION('ref_axis',(1.,0.,0.));
#10021=DIRECTION('center_axis',(0.,1.,0.));
#10022=DIRECTION('ref_axis',(1.,0.,0.));
#10023=DIRECTION('',(0.,1.,0.));
#10024=DIRECTION('center_axis',(0.,-1.,0.));
#10025=DIRECTION('ref_axis',(1.,0.,0.));
#10026=DIRECTION('center_axis',(0.,1.,0.));
#10027=DIRECTION('ref_axis',(1.,0.,0.));
#10028=DIRECTION('center_axis',(0.,1.,0.));
#10029=DIRECTION('ref_axis',(1.,0.,0.));
#10030=DIRECTION('',(0.,1.,0.));
#10031=DIRECTION('center_axis',(0.,-1.,0.));
#10032=DIRECTION('ref_axis',(1.,0.,0.));
#10033=DIRECTION('center_axis',(0.,1.,0.));
#10034=DIRECTION('ref_axis',(1.,0.,0.));
#10035=DIRECTION('center_axis',(0.,1.,0.));
#10036=DIRECTION('ref_axis',(1.,0.,0.));
#10037=DIRECTION('',(0.,1.,0.));
#10038=DIRECTION('center_axis',(0.,-1.,0.));
#10039=DIRECTION('ref_axis',(1.,0.,0.));
#10040=DIRECTION('center_axis',(0.,1.,0.));
#10041=DIRECTION('ref_axis',(1.,0.,0.));
#10042=DIRECTION('center_axis',(0.,1.,0.));
#10043=DIRECTION('ref_axis',(1.,0.,0.));
#10044=DIRECTION('',(0.,1.,0.));
#10045=DIRECTION('center_axis',(0.,-1.,0.));
#10046=DIRECTION('ref_axis',(1.,0.,0.));
#10047=DIRECTION('center_axis',(0.,0.,1.));
#10048=DIRECTION('ref_axis',(1.,0.,0.));
#10049=DIRECTION('center_axis',(0.,0.,1.));
#10050=DIRECTION('ref_axis',(1.,0.,0.));
#10051=DIRECTION('',(0.,0.,1.));
#10052=DIRECTION('center_axis',(0.,0.,-1.));
#10053=DIRECTION('ref_axis',(1.,0.,0.));
#10054=DIRECTION('center_axis',(0.,0.,1.));
#10055=DIRECTION('ref_axis',(1.,0.,0.));
#10056=DIRECTION('center_axis',(0.,0.,1.));
#10057=DIRECTION('ref_axis',(1.,0.,0.));
#10058=DIRECTION('',(0.,0.,1.));
#10059=DIRECTION('center_axis',(0.,0.,-1.));
#10060=DIRECTION('ref_axis',(1.,0.,0.));
#10061=DIRECTION('center_axis',(0.,0.,1.));
#10062=DIRECTION('ref_axis',(1.,0.,0.));
#10063=DIRECTION('center_axis',(0.,0.,1.));
#10064=DIRECTION('ref_axis',(1.,0.,0.));
#10065=DIRECTION('',(0.,0.,1.));
#10066=DIRECTION('center_axis',(0.,0.,-1.));
#10067=DIRECTION('ref_axis',(1.,0.,0.));
#10068=DIRECTION('center_axis',(0.,0.,1.));
#10069=DIRECTION('ref_axis',(1.,0.,0.));
#10070=DIRECTION('center_axis',(0.,0.,1.));
#10071=DIRECTION('ref_axis',(1.,0.,0.));
#10072=DIRECTION('',(0.,0.,1.));
#10073=DIRECTION('center_axis',(0.,0.,-1.));
#10074=DIRECTION('ref_axis',(1.,0.,0.));
#10075=DIRECTION('center_axis',(0.,0.,1.));
#10076=DIRECTION('ref_axis',(1.,0.,0.));
#10077=DIRECTION('center_axis',(0.,0.,1.));
#10078=DIRECTION('ref_axis',(1.,0.,0.));
#10079=DIRECTION('',(0.,0.,1.));
#10080=DIRECTION('center_axis',(0.,0.,-1.));
#10081=DIRECTION('ref_axis',(1.,0.,0.));
#10082=DIRECTION('center_axis',(0.,0.,1.));
#10083=DIRECTION('ref_axis',(1.,0.,0.));
#10084=DIRECTION('center_axis',(0.,0.,1.));
#10085=DIRECTION('ref_axis',(1.,0.,0.));
#10086=DIRECTION('center_axis',(0.,0.,1.));
#10087=DIRECTION('ref_axis',(1.,0.,0.));
#10088=DIRECTION('center_axis',(0.,0.,1.));
#10089=DIRECTION('ref_axis',(1.,0.,0.));
#10090=DIRECTION('',(0.,0.,1.));
#10091=DIRECTION('center_axis',(0.,1.,0.));
#10092=DIRECTION('ref_axis',(1.,0.,0.));
#10093=DIRECTION('center_axis',(0.,1.,0.));
#10094=DIRECTION('ref_axis',(1.,0.,0.));
#10095=DIRECTION('',(0.,1.,0.));
#10096=DIRECTION('center_axis',(0.,-1.,0.));
#10097=DIRECTION('ref_axis',(1.,0.,0.));
#10098=DIRECTION('center_axis',(0.,0.,1.));
#10099=DIRECTION('ref_axis',(1.,0.,0.));
#10100=DIRECTION('',(0.,0.,1.));
#10101=DIRECTION('center_axis',(0.,0.,1.));
#10102=DIRECTION('ref_axis',(1.,0.,0.));
#10103=DIRECTION('',(0.,0.,-1.));
#10104=DIRECTION('center_axis',(0.,0.,1.));
#10105=DIRECTION('ref_axis',(1.,0.,0.));
#10106=DIRECTION('center_axis',(0.,-1.,0.));
#10107=DIRECTION('ref_axis',(1.,0.,0.));
#10108=DIRECTION('',(-1.,0.,0.));
#10109=DIRECTION('',(0.,0.,1.));
#10110=DIRECTION('',(1.,0.,0.));
#10111=DIRECTION('',(0.,0.,1.));
#10112=DIRECTION('',(1.,0.,0.));
#10113=DIRECTION('',(0.,0.,1.));
#10114=DIRECTION('',(1.,0.,0.));
#10115=DIRECTION('center_axis',(0.,1.,0.));
#10116=DIRECTION('ref_axis',(1.,0.,0.));
#10117=DIRECTION('',(1.,0.,0.));
#10118=DIRECTION('center_axis',(0.,0.,1.));
#10119=DIRECTION('ref_axis',(1.,0.,0.));
#10120=DIRECTION('',(1.,0.,0.));
#10121=DIRECTION('',(0.,1.,0.));
#10122=DIRECTION('center_axis',(0.,0.,1.));
#10123=DIRECTION('ref_axis',(1.,0.,0.));
#10124=DIRECTION('',(0.,-1.,0.));
#10125=DIRECTION('',(1.,0.,0.));
#10126=DIRECTION('',(0.,1.,0.));
#10127=DIRECTION('',(-1.,0.,0.));
#10128=DIRECTION('',(-1.,0.,0.));
#10129=DIRECTION('',(0.,1.,0.));
#10130=DIRECTION('',(0.,-1.,0.));
#10131=DIRECTION('center_axis',(0.,1.,0.));
#10132=DIRECTION('ref_axis',(-1.,0.,0.));
#10133=DIRECTION('',(-1.,0.,0.));
#10134=DIRECTION('',(0.,0.,1.));
#10135=DIRECTION('',(0.,0.,1.));
#10136=DIRECTION('center_axis',(1.,0.,0.));
#10137=DIRECTION('ref_axis',(0.,1.,0.));
#10138=DIRECTION('',(0.,1.,0.));
#10139=DIRECTION('',(0.,0.,1.));
#10140=DIRECTION('center_axis',(0.,-1.,0.));
#10141=DIRECTION('ref_axis',(1.,0.,0.));
#10142=DIRECTION('',(1.,0.,0.));
#10143=DIRECTION('',(0.,0.,1.));
#10144=DIRECTION('center_axis',(-1.,0.,0.));
#10145=DIRECTION('ref_axis',(0.,-1.,0.));
#10146=DIRECTION('',(0.,-1.,0.));
#10147=DIRECTION('center_axis',(1.,0.,0.));
#10148=DIRECTION('ref_axis',(0.,1.,0.));
#10149=DIRECTION('',(0.,0.,1.));
#10150=DIRECTION('',(0.,-1.,0.));
#10151=DIRECTION('center_axis',(0.,1.,0.));
#10152=DIRECTION('ref_axis',(6.12323399573677E-17,0.,-1.));
#10153=DIRECTION('',(0.,1.,0.));
#10154=DIRECTION('',(0.,-1.,0.));
#10155=DIRECTION('center_axis',(0.,1.,0.));
#10156=DIRECTION('ref_axis',(1.,0.,0.));
#10157=DIRECTION('center_axis',(0.,1.,0.));
#10158=DIRECTION('ref_axis',(-1.,0.,0.));
#10159=DIRECTION('',(-1.,0.,0.));
#10160=DIRECTION('',(-1.,0.,0.));
#10161=DIRECTION('',(0.,0.,1.));
#10162=DIRECTION('',(-1.,0.,0.));
#10163=DIRECTION('',(0.,0.,1.));
#10164=DIRECTION('center_axis',(0.,0.,-1.));
#10165=DIRECTION('ref_axis',(-1.,0.,0.));
#10166=DIRECTION('center_axis',(0.,0.,-1.));
#10167=DIRECTION('ref_axis',(-1.,0.,0.));
#10168=DIRECTION('center_axis',(1.,0.,0.));
#10169=DIRECTION('ref_axis',(0.,1.,0.));
#10170=DIRECTION('',(0.,1.,0.));
#10171=DIRECTION('center_axis',(-1.,0.,0.));
#10172=DIRECTION('ref_axis',(0.,-1.,0.));
#10173=DIRECTION('',(0.,-1.,0.));
#10174=DIRECTION('center_axis',(0.,0.,1.));
#10175=DIRECTION('ref_axis',(1.,0.,0.));
#10176=DIRECTION('center_axis',(0.,0.,1.));
#10177=DIRECTION('ref_axis',(1.,0.,0.));
#12572=CARTESIAN_POINT('',(0.,0.,0.));
#12573=CARTESIAN_POINT('Origin',(-5.25982293614231,-0.9,14.8604204653858));
#12574=CARTESIAN_POINT('',(-5.48482293614231,-0.8,14.8604204653858));
#12575=CARTESIAN_POINT('Origin',(-5.25982293614231,-0.8,14.8604204653858));
#12576=CARTESIAN_POINT('',(-5.48482293614231,0.8,14.8604204653858));
#12577=CARTESIAN_POINT('',(-5.48482293614231,-0.9,14.8604204653858));
#12578=CARTESIAN_POINT('Origin',(-5.25982293614231,0.8,14.8604204653858));
#12579=CARTESIAN_POINT('Origin',(-1.13137084989848,-1.13137084989848,15.8));
#12580=CARTESIAN_POINT('',(-1.29637084989848,-1.13137084989848,15.8));
#12581=CARTESIAN_POINT('Origin',(-1.13137084989848,-1.13137084989848,15.8));
#12582=CARTESIAN_POINT('',(-1.29637084989848,-1.13137084989848,16.5));
#12583=CARTESIAN_POINT('',(-1.29637084989848,-1.13137084989848,15.8));
#12584=CARTESIAN_POINT('Origin',(-1.13137084989848,-1.13137084989848,16.5));
#12585=CARTESIAN_POINT('Origin',(-1.13137084989848,-1.13137084989848,15.8));
#12586=CARTESIAN_POINT('Origin',(-1.13137084989848,1.13137084989848,15.8));
#12587=CARTESIAN_POINT('',(-1.29637084989848,1.13137084989848,15.8));
#12588=CARTESIAN_POINT('Origin',(-1.13137084989848,1.13137084989848,15.8));
#12589=CARTESIAN_POINT('',(-1.29637084989848,1.13137084989848,16.5));
#12590=CARTESIAN_POINT('',(-1.29637084989848,1.13137084989848,15.8));
#12591=CARTESIAN_POINT('Origin',(-1.13137084989848,1.13137084989848,16.5));
#12592=CARTESIAN_POINT('Origin',(-1.13137084989848,1.13137084989848,15.8));
#12593=CARTESIAN_POINT('Origin',(1.13137084989848,1.13137084989848,15.8));
#12594=CARTESIAN_POINT('',(0.966370849898476,1.13137084989848,15.8));
#12595=CARTESIAN_POINT('Origin',(1.13137084989848,1.13137084989848,15.8));
#12596=CARTESIAN_POINT('',(0.966370849898476,1.13137084989848,16.5));
#12597=CARTESIAN_POINT('',(0.966370849898476,1.13137084989848,15.8));
#12598=CARTESIAN_POINT('Origin',(1.13137084989848,1.13137084989848,16.5));
#12599=CARTESIAN_POINT('Origin',(1.13137084989848,1.13137084989848,15.8));
#12600=CARTESIAN_POINT('Origin',(1.13137084989848,-1.13137084989848,15.8));
#12601=CARTESIAN_POINT('',(0.966370849898476,-1.13137084989848,15.8));
#12602=CARTESIAN_POINT('Origin',(1.13137084989848,-1.13137084989848,15.8));
#12603=CARTESIAN_POINT('',(0.966370849898476,-1.13137084989848,16.5));
#12604=CARTESIAN_POINT('',(0.966370849898476,-1.13137084989848,15.8));
#12605=CARTESIAN_POINT('Origin',(1.13137084989848,-1.13137084989848,16.5));
#12606=CARTESIAN_POINT('Origin',(1.13137084989848,-1.13137084989848,15.8));
#12607=CARTESIAN_POINT('Origin',(-5.23743686707646,-0.9,9.76256313292354));
#12608=CARTESIAN_POINT('',(-5.40243686707646,-0.8,9.76256313292354));
#12609=CARTESIAN_POINT('Origin',(-5.23743686707646,-0.8,9.76256313292354));
#12610=CARTESIAN_POINT('',(-5.40243686707646,0.8,9.76256313292354));
#12611=CARTESIAN_POINT('',(-5.40243686707646,-0.9,9.76256313292354));
#12612=CARTESIAN_POINT('Origin',(-5.23743686707646,0.8,9.76256313292354));
#12613=CARTESIAN_POINT('Origin',(-5.23743686707646,-0.9,12.2374368670765));
#12614=CARTESIAN_POINT('',(-5.40243686707646,-0.8,12.2374368670765));
#12615=CARTESIAN_POINT('Origin',(-5.23743686707646,-0.8,12.2374368670765));
#12616=CARTESIAN_POINT('',(-5.40243686707646,0.8,12.2374368670765));
#12617=CARTESIAN_POINT('',(-5.40243686707646,-0.9,12.2374368670765));
#12618=CARTESIAN_POINT('Origin',(-5.23743686707646,0.8,12.2374368670765));
#12619=CARTESIAN_POINT('Origin',(-2.76256313292354,-0.9,12.2374368670765));
#12620=CARTESIAN_POINT('',(-2.92756313292354,-0.8,12.2374368670765));
#12621=CARTESIAN_POINT('Origin',(-2.76256313292354,-0.8,12.2374368670765));
#12622=CARTESIAN_POINT('',(-2.92756313292354,0.8,12.2374368670765));
#12623=CARTESIAN_POINT('',(-2.92756313292354,-0.9,12.2374368670765));
#12624=CARTESIAN_POINT('Origin',(-2.76256313292354,0.8,12.2374368670765));
#12625=CARTESIAN_POINT('Origin',(-2.76256313292354,-0.9,9.76256313292354));
#12626=CARTESIAN_POINT('',(-2.92756313292354,-0.8,9.76256313292354));
#12627=CARTESIAN_POINT('Origin',(-2.76256313292354,-0.8,9.76256313292354));
#12628=CARTESIAN_POINT('',(-2.92756313292354,0.8,9.76256313292354));
#12629=CARTESIAN_POINT('',(-2.92756313292354,-0.9,9.76256313292354));
#12630=CARTESIAN_POINT('Origin',(-2.76256313292354,0.8,9.76256313292354));
#12631=CARTESIAN_POINT('Origin',(-6.,-1.4,0.9));
#12632=CARTESIAN_POINT('',(-6.275,-1.4,1.));
#12633=CARTESIAN_POINT('Origin',(-6.,-1.4,1.));
#12634=CARTESIAN_POINT('',(-6.275,-1.4,1.8));
#12635=CARTESIAN_POINT('',(-6.275,-1.4,0.9));
#12636=CARTESIAN_POINT('Origin',(-6.,-1.4,1.8));
#12637=CARTESIAN_POINT('Origin',(-8.5,1.4,0.9));
#12638=CARTESIAN_POINT('',(-8.775,1.4,1.));
#12639=CARTESIAN_POINT('Origin',(-8.5,1.4,1.));
#12640=CARTESIAN_POINT('',(-8.775,1.4,1.8));
#12641=CARTESIAN_POINT('',(-8.775,1.4,0.9));
#12642=CARTESIAN_POINT('Origin',(-8.5,1.4,1.8));
#12643=CARTESIAN_POINT('Origin',(-8.5,-1.4,0.9));
#12644=CARTESIAN_POINT('',(-8.775,-1.4,1.));
#12645=CARTESIAN_POINT('Origin',(-8.5,-1.4,1.));
#12646=CARTESIAN_POINT('',(-8.775,-1.4,1.8));
#12647=CARTESIAN_POINT('',(-8.775,-1.4,0.9));
#12648=CARTESIAN_POINT('Origin',(-8.5,-1.4,1.8));
#12649=CARTESIAN_POINT('Origin',(-6.,1.4,0.9));
#12650=CARTESIAN_POINT('',(-6.275,1.4,1.));
#12651=CARTESIAN_POINT('Origin',(-6.,1.4,1.));
#12652=CARTESIAN_POINT('',(-6.275,1.4,1.8));
#12653=CARTESIAN_POINT('',(-6.275,1.4,0.9));
#12654=CARTESIAN_POINT('Origin',(-6.,1.4,1.8));
#12655=CARTESIAN_POINT('Origin',(0.,0.,12.5));
#12656=CARTESIAN_POINT('',(-1.05,-1.28587913910472E-16,12.5));
#12657=CARTESIAN_POINT('Origin',(0.,0.,12.5));
#12658=CARTESIAN_POINT('',(-1.05,1.28587913910472E-16,16.5));
#12659=CARTESIAN_POINT('',(-1.05,-1.28587913910472E-16,12.5));
#12660=CARTESIAN_POINT('Origin',(0.,0.,16.5));
#12661=CARTESIAN_POINT('Origin',(0.,0.,12.5));
#12662=CARTESIAN_POINT('',(-0.625,-7.65404249467096E-17,12.5));
#12663=CARTESIAN_POINT('Origin',(0.,0.,12.5));
#12664=CARTESIAN_POINT('Origin',(0.,0.,11.9));
#12665=CARTESIAN_POINT('',(-0.625,-7.65404249467096E-17,12.));
#12666=CARTESIAN_POINT('Origin',(0.,0.,12.));
#12667=CARTESIAN_POINT('',(-0.625,-7.65404249467096E-17,11.9));
#12668=CARTESIAN_POINT('Origin',(-4.,-0.9,11.));
#12669=CARTESIAN_POINT('',(-5.5,-0.8,11.));
#12670=CARTESIAN_POINT('Origin',(-4.,-0.8,11.));
#12671=CARTESIAN_POINT('',(-5.5,0.8,11.));
#12672=CARTESIAN_POINT('',(-5.5,-0.9,11.));
#12673=CARTESIAN_POINT('Origin',(-4.,0.8,11.));
#12674=CARTESIAN_POINT('Origin',(0.,0.,12.));
#12675=CARTESIAN_POINT('',(-1.83303027798234,-0.8,12.));
#12676=CARTESIAN_POINT('',(-1.83303027798234,-0.8,16.5));
#12677=CARTESIAN_POINT('',(-1.83303027798234,-0.8,12.));
#12678=CARTESIAN_POINT('',(-1.83303027798234,0.8,12.));
#12679=CARTESIAN_POINT('Origin',(0.,0.,12.));
#12680=CARTESIAN_POINT('',(-1.83303027798234,0.8,16.5));
#12681=CARTESIAN_POINT('',(-1.83303027798234,0.8,12.));
#12682=CARTESIAN_POINT('Origin',(0.,0.,16.5));
#12683=CARTESIAN_POINT('Origin',(-8.,-0.8,1.));
#12684=CARTESIAN_POINT('',(-6.5,-0.8,16.5));
#12685=CARTESIAN_POINT('',(1.5,-0.8,16.5));
#12686=CARTESIAN_POINT('',(-6.5,-0.8,17.5));
#12687=CARTESIAN_POINT('',(-6.5,-0.8,1.));
#12688=CARTESIAN_POINT('',(-8.,-0.8,17.5));
#12689=CARTESIAN_POINT('',(-8.,-0.8,17.5));
#12690=CARTESIAN_POINT('',(-8.,-0.8,1.8));
#12691=CARTESIAN_POINT('',(-8.,-0.8,1.));
#12692=CARTESIAN_POINT('',(-6.5,-0.8,1.8));
#12693=CARTESIAN_POINT('',(-7.625,-0.8,1.8));
#12694=CARTESIAN_POINT('',(-6.5,-0.8,12.));
#12695=CARTESIAN_POINT('',(-6.5,-0.8,1.));
#12696=CARTESIAN_POINT('',(-5.95959179422654,-0.8,12.));
#12697=CARTESIAN_POINT('',(-8.,-0.8,12.));
#12698=CARTESIAN_POINT('',(-2.04040820577346,-0.8,12.));
#12699=CARTESIAN_POINT('Origin',(-4.,-0.8,11.));
#12700=CARTESIAN_POINT('',(-8.,-0.8,12.));
#12701=CARTESIAN_POINT('Origin',(-8.,-0.8,16.5));
#12702=CARTESIAN_POINT('',(-6.5,0.8,16.5));
#12703=CARTESIAN_POINT('',(1.5,0.8,16.5));
#12704=CARTESIAN_POINT('',(-6.5,-0.8,16.5));
#12705=CARTESIAN_POINT('Origin',(-7.25,0.,1.8));
#12706=CARTESIAN_POINT('',(-9.,2.,1.8));
#12707=CARTESIAN_POINT('',(-9.,-2.,1.8));
#12708=CARTESIAN_POINT('',(-9.,2.,1.8));
#12709=CARTESIAN_POINT('',(-5.5,-2.,1.8));
#12710=CARTESIAN_POINT('',(-9.,-2.,1.8));
#12711=CARTESIAN_POINT('',(-5.5,2.,1.8));
#12712=CARTESIAN_POINT('',(-5.5,-2.,1.8));
#12713=CARTESIAN_POINT('',(-5.5,2.,1.8));
#12714=CARTESIAN_POINT('',(-6.5,0.8,1.8));
#12715=CARTESIAN_POINT('',(-8.,0.8,1.8));
#12716=CARTESIAN_POINT('',(-6.875,0.8,1.8));
#12717=CARTESIAN_POINT('',(-6.5,-0.4,1.8));
#12718=CARTESIAN_POINT('',(-8.,0.4,1.8));
#12719=CARTESIAN_POINT('Origin',(-5.5,2.,1.));
#12720=CARTESIAN_POINT('',(-5.5,2.,1.));
#12721=CARTESIAN_POINT('',(-9.,2.,1.));
#12722=CARTESIAN_POINT('',(-5.5,2.,1.));
#12723=CARTESIAN_POINT('',(-9.,2.,1.));
#12724=CARTESIAN_POINT('',(-5.5,2.,1.));
#12725=CARTESIAN_POINT('Origin',(-5.5,-2.,1.));
#12726=CARTESIAN_POINT('',(-5.5,-2.,1.));
#12727=CARTESIAN_POINT('',(-5.5,-2.,1.));
#12728=CARTESIAN_POINT('',(-5.5,-2.,1.));
#12729=CARTESIAN_POINT('Origin',(-9.,-2.,1.));
#12730=CARTESIAN_POINT('',(-9.,-2.,1.));
#12731=CARTESIAN_POINT('',(-9.,-2.,1.));
#12732=CARTESIAN_POINT('',(-9.,-2.,1.));
#12733=CARTESIAN_POINT('Origin',(-9.,2.,1.));
#12734=CARTESIAN_POINT('',(-9.,2.,1.));
#12735=CARTESIAN_POINT('Origin',(-6.5,-0.8,1.));
#12736=CARTESIAN_POINT('',(-6.5,0.8,12.));
#12737=CARTESIAN_POINT('',(-6.5,0.8,1.));
#12738=CARTESIAN_POINT('',(-6.5,-0.8,12.));
#12739=CARTESIAN_POINT('Origin',(-4.,-0.8,11.));
#12740=CARTESIAN_POINT('',(-2.04040820577346,0.8,12.));
#12741=CARTESIAN_POINT('',(-2.04040820577346,-0.8,12.));
#12742=CARTESIAN_POINT('',(-5.95959179422654,0.8,12.));
#12743=CARTESIAN_POINT('',(-5.95959179422654,-0.8,12.));
#12744=CARTESIAN_POINT('Origin',(-4.,0.8,11.));
#12745=CARTESIAN_POINT('Origin',(-6.5,0.8,1.));
#12746=CARTESIAN_POINT('',(-8.,0.8,12.));
#12747=CARTESIAN_POINT('',(-8.,0.8,12.));
#12748=CARTESIAN_POINT('',(-8.,0.8,17.5));
#12749=CARTESIAN_POINT('',(-8.,0.8,1.));
#12750=CARTESIAN_POINT('',(-6.5,0.8,17.5));
#12751=CARTESIAN_POINT('',(-6.5,0.8,17.5));
#12752=CARTESIAN_POINT('',(-6.5,0.8,1.));
#12753=CARTESIAN_POINT('Origin',(1.5,-0.8,12.));
#12754=CARTESIAN_POINT('Origin',(1.5,-0.8,12.));
#12755=CARTESIAN_POINT('Origin',(-6.5,-0.8,1.));
#12756=CARTESIAN_POINT('',(-6.5,-0.8,17.5));
#12757=CARTESIAN_POINT('Origin',(-8.,0.8,1.));
#12758=CARTESIAN_POINT('',(-8.,0.8,17.5));
#12759=CARTESIAN_POINT('Origin',(-7.25,0.,17.5));
#12760=CARTESIAN_POINT('Origin',(-7.25,0.,1.));
#15119=UNCERTAINTY_MEASURE_WITH_UNIT(LENGTH_MEASURE(0.001),#15213,
'DISTANCE_ACCURACY_VALUE',
'Maximum model space distance between geometric entities at asserted c
onnectivities');
#15162=UNCERTAINTY_MEASURE_WITH_UNIT(LENGTH_MEASURE(0.001),#15213,
'DISTANCE_ACCURACY_VALUE',
'Maximum model space distance between geometric entities at asserted c
onnectivities');
#15169=(
GEOMETRIC_REPRESENTATION_CONTEXT(3)
GLOBAL_UNCERTAINTY_ASSIGNED_CONTEXT((#15119))
GLOBAL_UNIT_ASSIGNED_CONTEXT((#15213,#15215,#15216))
REPRESENTATION_CONTEXT('','3D')
);
#15212=(
GEOMETRIC_REPRESENTATION_CONTEXT(3)
GLOBAL_UNCERTAINTY_ASSIGNED_CONTEXT((#15162))
GLOBAL_UNIT_ASSIGNED_CONTEXT((#15213,#15215,#15216))
REPRESENTATION_CONTEXT('','3D')
);
#15213=(
LENGTH_UNIT()
NAMED_UNIT(*)
SI_UNIT(.CENTI.,.METRE.)
);
#15215=(
NAMED_UNIT(*)
PLANE_ANGLE_UNIT()
SI_UNIT($,.RADIAN.)
);
#15216=(
NAMED_UNIT(*)
SI_UNIT($,.STERADIAN.)
SOLID_ANGLE_UNIT()
);
#15223=SHAPE_DEFINITION_REPRESENTATION(#15272,#15407);
#15272=PRODUCT_DEFINITION_SHAPE('',$,#15457);
#15407=SHAPE_REPRESENTATION('',(#8841),#15169);
#15450=PRODUCT_DEFINITION_CONTEXT('part definition',#15599,'design');
#15457=PRODUCT_DEFINITION('Bearing frame','Bearing frame',#15506,#15450);
#15506=PRODUCT_DEFINITION_FORMATION('',$,#15607);
#15599=APPLICATION_CONTEXT(
'Core Data for Automotive Mechanical Design Process');
#15600=PRODUCT_CONTEXT('part definition',#15599,'mechanical');
#15607=PRODUCT('Bearing frame','Bearing frame','Bearing frame',(#15600));
#15713=COLOUR_RGB('Grey',0.48,0.52,0.57);
#15714=FILL_AREA_STYLE_COLOUR('',#15713);
#15715=FILL_AREA_STYLE('',(#15714));
#15716=SURFACE_STYLE_FILL_AREA(#15715);
#15717=SURFACE_SIDE_STYLE('',(#15716));
#15718=SURFACE_STYLE_USAGE(.BOTH.,#15717);
#15719=PRESENTATION_STYLE_ASSIGNMENT((#15718));
ENDSEC;
END-ISO-10303-21;
